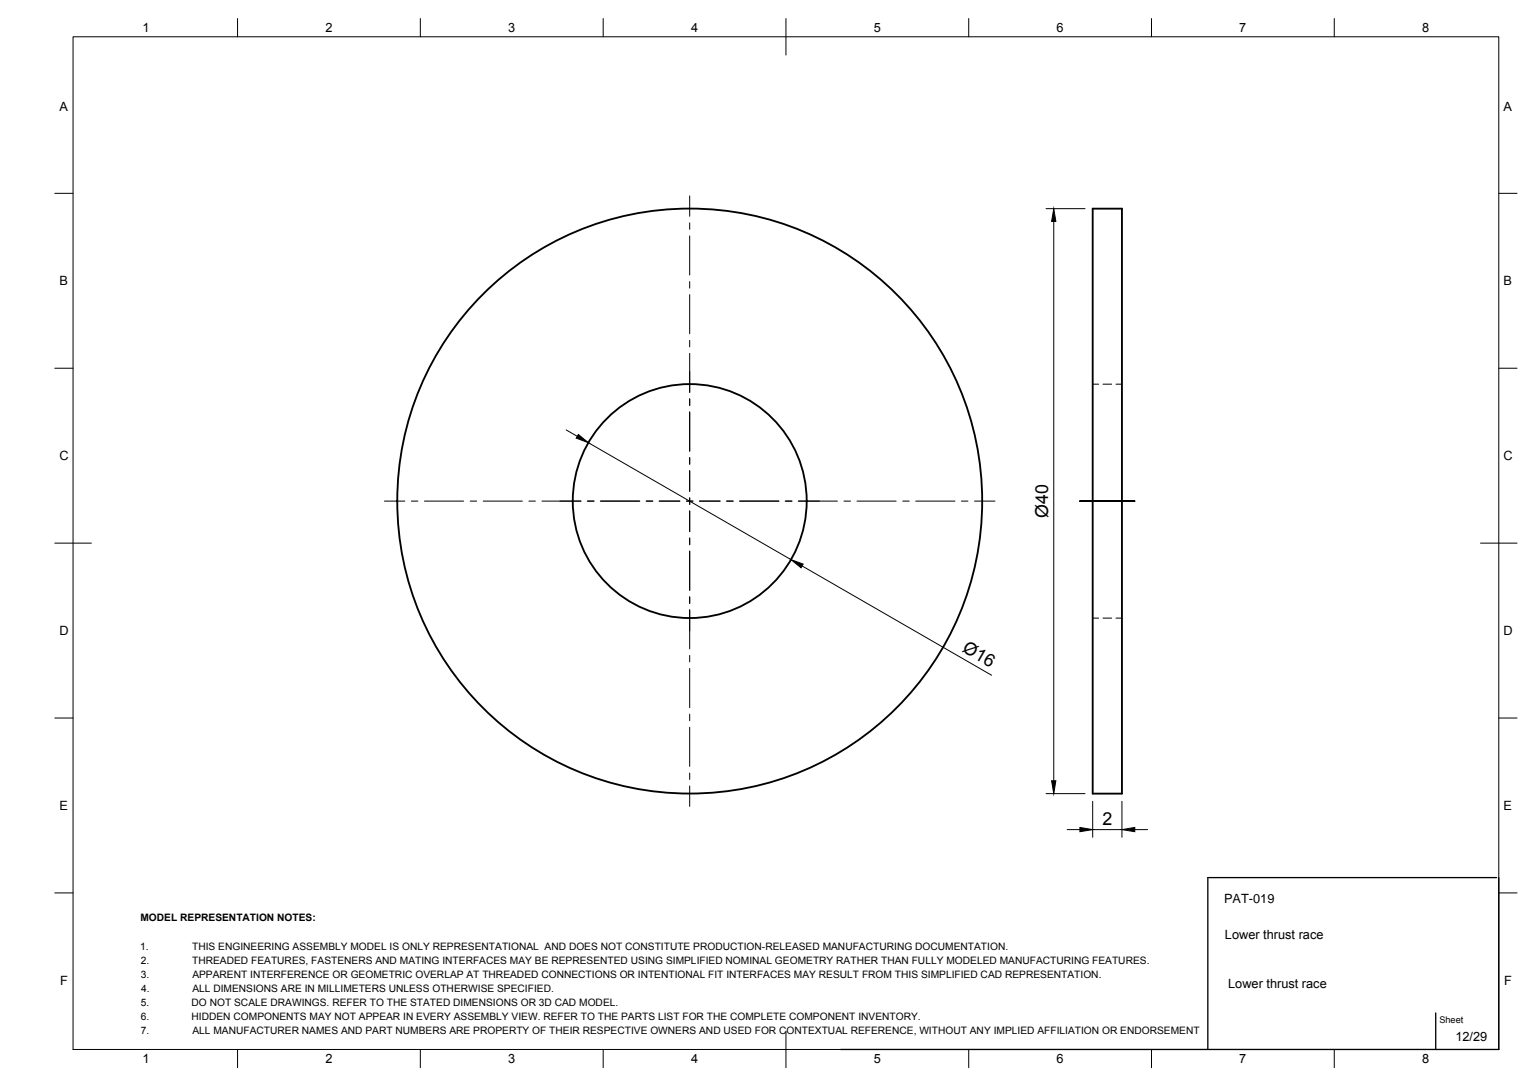
ISO-10303-21;
HEADER;
/* Generated by software containing ST-Developer
 * from STEP Tools, Inc. (www.steptools.com) 
 */

FILE_DESCRIPTION(
/* description */ ('Caster wheel assembly'),
/* implementation_level */ '2;1');

FILE_NAME(
/* name */ 'Lower thrust race.step',
/* time_stamp */ '2026-10-28T03:23:56-07:00',
/* author */ (''),
/* organization */ (''),
/* preprocessor_version */ 'ST-DEVELOPER v20.2',
/* originating_system */ 'Autodesk Translation Framework v15.17.0.0',
/* authorisation */ '');

FILE_SCHEMA (('AUTOMOTIVE_DESIGN { 1 0 10303 214 3 1 1 }'));
ENDSEC;

DATA;
#10=MECHANICAL_DESIGN_GEOMETRIC_PRESENTATION_REPRESENTATION('',(#229),#5385);
#185=SHAPE_REPRESENTATION_RELATIONSHIP('SRR','None',#5481,#207);
#207=ADVANCED_BREP_SHAPE_REPRESENTATION('',(#259),#5368);
#229=STYLED_ITEM('',(#5665),#259);
#259=MANIFOLD_SOLID_BREP('Body1',#2656);
#303=FACE_BOUND('',#672,.T.);
#304=FACE_BOUND('',#674,.T.);
#371=PLANE('',#3041);
#372=PLANE('',#3042);
#479=FACE_OUTER_BOUND('',#669,.T.);
#480=FACE_OUTER_BOUND('',#670,.T.);
#481=FACE_OUTER_BOUND('',#671,.T.);
#482=FACE_OUTER_BOUND('',#673,.T.);
#669=EDGE_LOOP('',(#2030,#2031,#2032,#2033));
#670=EDGE_LOOP('',(#2034,#2035,#2036,#2037));
#671=EDGE_LOOP('',(#2038));
#672=EDGE_LOOP('',(#2039));
#673=EDGE_LOOP('',(#2040));
#674=EDGE_LOOP('',(#2041));
#883=LINE('',#4508,#1017);
#884=LINE('',#4514,#1018);
#1017=VECTOR('',#3606,0.8);
#1018=VECTOR('',#3613,2.);
#1115=CIRCLE('',#3036,0.8);
#1116=CIRCLE('',#3037,0.8);
#1117=CIRCLE('',#3039,2.);
#1118=CIRCLE('',#3040,2.);
#1318=VERTEX_POINT('',#4505);
#1319=VERTEX_POINT('',#4507);
#1320=VERTEX_POINT('',#4511);
#1321=VERTEX_POINT('',#4513);
#1583=EDGE_CURVE('',#1318,#1318,#1115,.T.);
#1584=EDGE_CURVE('',#1318,#1319,#883,.T.);
#1585=EDGE_CURVE('',#1319,#1319,#1116,.T.);
#1586=EDGE_CURVE('',#1320,#1320,#1117,.T.);
#1587=EDGE_CURVE('',#1320,#1321,#884,.T.);
#1588=EDGE_CURVE('',#1321,#1321,#1118,.T.);
#2030=ORIENTED_EDGE('',*,*,#1583,.F.);
#2031=ORIENTED_EDGE('',*,*,#1584,.T.);
#2032=ORIENTED_EDGE('',*,*,#1585,.T.);
#2033=ORIENTED_EDGE('',*,*,#1584,.F.);
#2034=ORIENTED_EDGE('',*,*,#1586,.F.);
#2035=ORIENTED_EDGE('',*,*,#1587,.T.);
#2036=ORIENTED_EDGE('',*,*,#1588,.T.);
#2037=ORIENTED_EDGE('',*,*,#1587,.F.);
#2038=ORIENTED_EDGE('',*,*,#1586,.T.);
#2039=ORIENTED_EDGE('',*,*,#1583,.T.);
#2040=ORIENTED_EDGE('',*,*,#1588,.F.);
#2041=ORIENTED_EDGE('',*,*,#1585,.F.);
#2446=CYLINDRICAL_SURFACE('',#3035,0.8);
#2447=CYLINDRICAL_SURFACE('',#3038,2.);
#2539=ADVANCED_FACE('',(#479),#2446,.F.);
#2540=ADVANCED_FACE('',(#480),#2447,.T.);
#2541=ADVANCED_FACE('',(#481,#303),#371,.T.);
#2542=ADVANCED_FACE('',(#482,#304),#372,.F.);
#2656=CLOSED_SHELL('',(#2539,#2540,#2541,#2542));
#3034=AXIS2_PLACEMENT_3D('',#4503,#3600,#3601);
#3035=AXIS2_PLACEMENT_3D('',#4504,#3602,#3603);
#3036=AXIS2_PLACEMENT_3D('',#4506,#3604,#3605);
#3037=AXIS2_PLACEMENT_3D('',#4509,#3607,#3608);
#3038=AXIS2_PLACEMENT_3D('',#4510,#3609,#3610);
#3039=AXIS2_PLACEMENT_3D('',#4512,#3611,#3612);
#3040=AXIS2_PLACEMENT_3D('',#4515,#3614,#3615);
#3041=AXIS2_PLACEMENT_3D('',#4516,#3616,#3617);
#3042=AXIS2_PLACEMENT_3D('',#4517,#3618,#3619);
#3600=DIRECTION('axis',(0.,0.,1.));
#3601=DIRECTION('refdir',(1.,0.,0.));
#3602=DIRECTION('center_axis',(0.,0.,1.));
#3603=DIRECTION('ref_axis',(1.,0.,0.));
#3604=DIRECTION('center_axis',(0.,0.,-1.));
#3605=DIRECTION('ref_axis',(1.,0.,0.));
#3606=DIRECTION('',(0.,0.,-1.));
#3607=DIRECTION('center_axis',(0.,0.,-1.));
#3608=DIRECTION('ref_axis',(1.,0.,0.));
#3609=DIRECTION('center_axis',(0.,0.,1.));
#3610=DIRECTION('ref_axis',(1.,0.,0.));
#3611=DIRECTION('center_axis',(0.,0.,1.));
#3612=DIRECTION('ref_axis',(1.,0.,0.));
#3613=DIRECTION('',(0.,0.,-1.));
#3614=DIRECTION('center_axis',(0.,0.,1.));
#3615=DIRECTION('ref_axis',(1.,0.,0.));
#3616=DIRECTION('center_axis',(0.,0.,1.));
#3617=DIRECTION('ref_axis',(1.,0.,0.));
#3618=DIRECTION('center_axis',(0.,0.,1.));
#3619=DIRECTION('ref_axis',(1.,0.,0.));
#4503=CARTESIAN_POINT('',(0.,0.,0.));
#4504=CARTESIAN_POINT('Origin',(-2.,0.,9.3));
#4505=CARTESIAN_POINT('',(-2.8,-9.79717439317883E-17,9.5));
#4506=CARTESIAN_POINT('Origin',(-2.,0.,9.5));
#4507=CARTESIAN_POINT('',(-2.8,-9.79717439317883E-17,9.3));
#4508=CARTESIAN_POINT('',(-2.8,-9.79717439317883E-17,9.3));
#4509=CARTESIAN_POINT('Origin',(-2.,0.,9.3));
#4510=CARTESIAN_POINT('Origin',(-2.,0.,9.3));
#4511=CARTESIAN_POINT('',(-4.,-2.44929359829471E-16,9.5));
#4512=CARTESIAN_POINT('Origin',(-2.,0.,9.5));
#4513=CARTESIAN_POINT('',(-4.,-2.44929359829471E-16,9.3));
#4514=CARTESIAN_POINT('',(-4.,-2.44929359829471E-16,9.3));
#4515=CARTESIAN_POINT('Origin',(-2.,0.,9.3));
#4516=CARTESIAN_POINT('Origin',(-2.,0.,9.5));
#4517=CARTESIAN_POINT('Origin',(-2.,0.,9.3));
#5340=UNCERTAINTY_MEASURE_WITH_UNIT(LENGTH_MEASURE(0.001),#5386,
'DISTANCE_ACCURACY_VALUE',
'Maximum model space distance between geometric entities at asserted c
onnectivities');
#5357=UNCERTAINTY_MEASURE_WITH_UNIT(LENGTH_MEASURE(0.001),#5386,
'DISTANCE_ACCURACY_VALUE',
'Maximum model space distance between geometric entities at asserted c
onnectivities');
#5368=(
GEOMETRIC_REPRESENTATION_CONTEXT(3)
GLOBAL_UNCERTAINTY_ASSIGNED_CONTEXT((#5340))
GLOBAL_UNIT_ASSIGNED_CONTEXT((#5386,#5388,#5389))
REPRESENTATION_CONTEXT('','3D')
);
#5385=(
GEOMETRIC_REPRESENTATION_CONTEXT(3)
GLOBAL_UNCERTAINTY_ASSIGNED_CONTEXT((#5357))
GLOBAL_UNIT_ASSIGNED_CONTEXT((#5386,#5388,#5389))
REPRESENTATION_CONTEXT('','3D')
);
#5386=(
LENGTH_UNIT()
NAMED_UNIT(*)
SI_UNIT(.CENTI.,.METRE.)
);
#5388=(
NAMED_UNIT(*)
PLANE_ANGLE_UNIT()
SI_UNIT($,.RADIAN.)
);
#5389=(
NAMED_UNIT(*)
SI_UNIT($,.STERADIAN.)
SOLID_ANGLE_UNIT()
);
#5400=SHAPE_DEFINITION_REPRESENTATION(#5432,#5481);
#5432=PRODUCT_DEFINITION_SHAPE('',$,#5509);
#5481=SHAPE_REPRESENTATION('',(#3034),#5368);
#5498=PRODUCT_DEFINITION_CONTEXT('part definition',#5581,'design');
#5509=PRODUCT_DEFINITION('Lower thrust race','Lower thrust race',#5536,
#5498);
#5536=PRODUCT_DEFINITION_FORMATION('',$,#5593);
#5581=APPLICATION_CONTEXT(
'Core Data for Automotive Mechanical Design Process');
#5582=PRODUCT_CONTEXT('part definition',#5581,'mechanical');
#5593=PRODUCT('Lower thrust race','Lower thrust race',
'Lower thrust race',(#5582));
#5659=COLOUR_RGB('Sky Blue',0.24,0.69,0.87);
#5660=FILL_AREA_STYLE_COLOUR('',#5659);
#5661=FILL_AREA_STYLE('',(#5660));
#5662=SURFACE_STYLE_FILL_AREA(#5661);
#5663=SURFACE_SIDE_STYLE('',(#5662));
#5664=SURFACE_STYLE_USAGE(.BOTH.,#5663);
#5665=PRESENTATION_STYLE_ASSIGNMENT((#5664));
ENDSEC;
END-ISO-10303-21;
